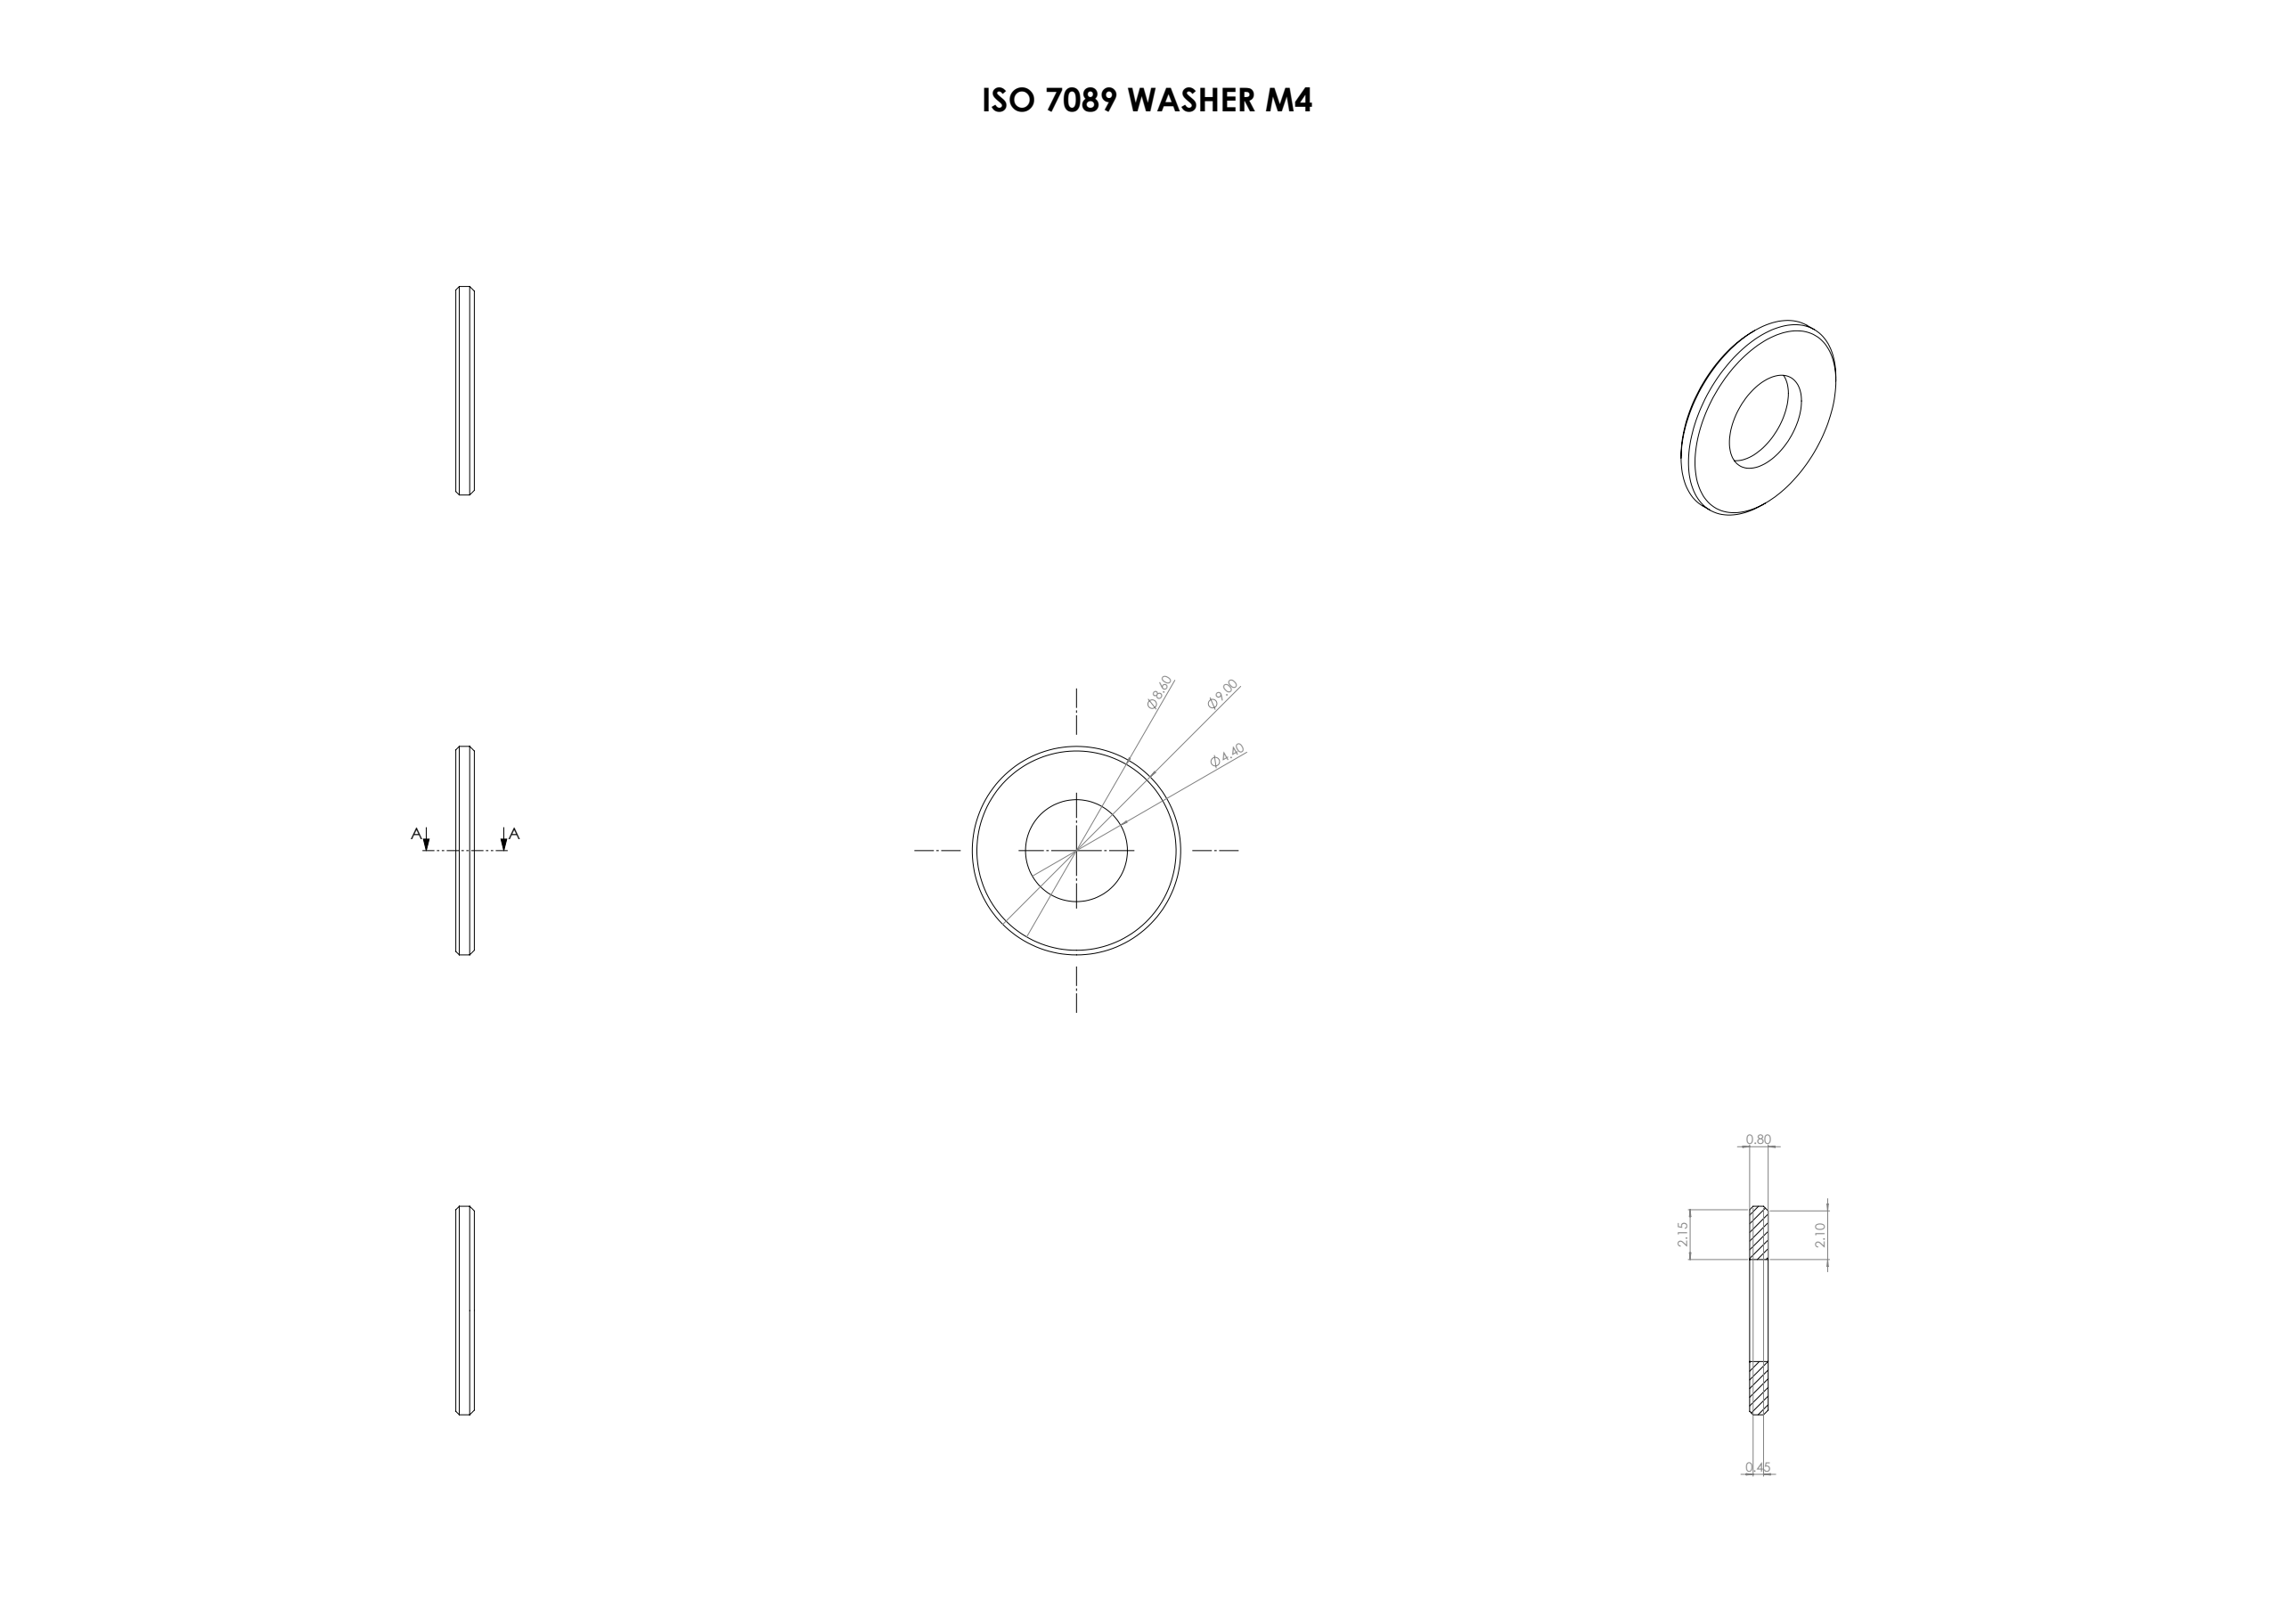
ISO-10303-21;
HEADER;
/* Generated by software containing ST-Developer
 * from STEP Tools, Inc. (www.steptools.com) 
 */

FILE_DESCRIPTION(
/* description */ (''),
/* implementation_level */ '2;1');

FILE_NAME(
/* name */ '12_ISO_7089_Washer_M4.step',
/* time_stamp */ '2026-10-21T02:01:14-07:00',
/* author */ (''),
/* organization */ (''),
/* preprocessor_version */ 'ST-DEVELOPER v20.2',
/* originating_system */ 'Autodesk Translation Framework v15.15.0.0',
/* authorisation */ '');

FILE_SCHEMA (('AUTOMOTIVE_DESIGN { 1 0 10303 214 3 1 1 }'));
ENDSEC;

DATA;
#10=MECHANICAL_DESIGN_GEOMETRIC_PRESENTATION_REPRESENTATION('',(#624),#37181);
#598=SHAPE_REPRESENTATION_RELATIONSHIP('SRR','None',#37248,#611);
#611=ADVANCED_BREP_SHAPE_REPRESENTATION('',(#637),#37178);
#624=STYLED_ITEM('',(#37380),#637);
#637=MANIFOLD_SOLID_BREP('Body1',#14786);
#684=FACE_BOUND('',#3017,.T.);
#685=FACE_BOUND('',#3020,.T.);
#910=CYLINDRICAL_SURFACE('',#16004,4.5);
#911=CYLINDRICAL_SURFACE('',#16008,2.2);
#1258=CIRCLE('',#16001,4.3);
#1259=CIRCLE('',#16002,4.5);
#1260=CIRCLE('',#16003,4.5);
#1261=CIRCLE('',#16005,4.5);
#1262=CIRCLE('',#16007,2.2);
#1263=CIRCLE('',#16009,2.2);
#1264=CIRCLE('',#16011,4.35);
#1360=CONICAL_SURFACE('',#16000,4.4,0.785398163397449);
#1361=CONICAL_SURFACE('',#16012,4.425,0.785398163397451);
#2130=FACE_OUTER_BOUND('',#3014,.T.);
#2131=FACE_OUTER_BOUND('',#3015,.T.);
#2132=FACE_OUTER_BOUND('',#3016,.T.);
#2133=FACE_OUTER_BOUND('',#3018,.T.);
#2134=FACE_OUTER_BOUND('',#3019,.T.);
#2135=FACE_OUTER_BOUND('',#3021,.T.);
#3014=EDGE_LOOP('',(#13047,#13048,#13049,#13050,#13051));
#3015=EDGE_LOOP('',(#13052,#13053,#13054,#13055,#13056));
#3016=EDGE_LOOP('',(#13057));
#3017=EDGE_LOOP('',(#13058));
#3018=EDGE_LOOP('',(#13059,#13060,#13061,#13062));
#3019=EDGE_LOOP('',(#13063));
#3020=EDGE_LOOP('',(#13064));
#3021=EDGE_LOOP('',(#13065,#13066,#13067,#13068));
#4371=LINE('',#34284,#5610);
#4372=LINE('',#34290,#5611);
#4373=LINE('',#34297,#5612);
#4374=LINE('',#34303,#5613);
#5610=VECTOR('',#19431,4.4);
#5611=VECTOR('',#19438,4.5);
#5612=VECTOR('',#19447,2.2);
#5613=VECTOR('',#19456,4.425);
#6891=VERTEX_POINT('',#34281);
#6892=VERTEX_POINT('',#34283);
#6893=VERTEX_POINT('',#34285);
#6894=VERTEX_POINT('',#34289);
#6895=VERTEX_POINT('',#34293);
#6896=VERTEX_POINT('',#34296);
#6897=VERTEX_POINT('',#34300);
#8965=EDGE_CURVE('',#6891,#6891,#1258,.T.);
#8966=EDGE_CURVE('',#6891,#6892,#4371,.T.);
#8967=EDGE_CURVE('',#6892,#6893,#1259,.T.);
#8968=EDGE_CURVE('',#6893,#6892,#1260,.T.);
#8969=EDGE_CURVE('',#6893,#6894,#4372,.T.);
#8970=EDGE_CURVE('',#6894,#6894,#1261,.T.);
#8971=EDGE_CURVE('',#6895,#6895,#1262,.T.);
#8972=EDGE_CURVE('',#6895,#6896,#4373,.T.);
#8973=EDGE_CURVE('',#6896,#6896,#1263,.T.);
#8974=EDGE_CURVE('',#6897,#6897,#1264,.T.);
#8975=EDGE_CURVE('',#6894,#6897,#4374,.T.);
#13047=ORIENTED_EDGE('',*,*,#8965,.T.);
#13048=ORIENTED_EDGE('',*,*,#8966,.T.);
#13049=ORIENTED_EDGE('',*,*,#8967,.T.);
#13050=ORIENTED_EDGE('',*,*,#8968,.T.);
#13051=ORIENTED_EDGE('',*,*,#8966,.F.);
#13052=ORIENTED_EDGE('',*,*,#8967,.F.);
#13053=ORIENTED_EDGE('',*,*,#8968,.F.);
#13054=ORIENTED_EDGE('',*,*,#8969,.T.);
#13055=ORIENTED_EDGE('',*,*,#8970,.T.);
#13056=ORIENTED_EDGE('',*,*,#8969,.F.);
#13057=ORIENTED_EDGE('',*,*,#8965,.F.);
#13058=ORIENTED_EDGE('',*,*,#8971,.F.);
#13059=ORIENTED_EDGE('',*,*,#8971,.T.);
#13060=ORIENTED_EDGE('',*,*,#8972,.T.);
#13061=ORIENTED_EDGE('',*,*,#8973,.F.);
#13062=ORIENTED_EDGE('',*,*,#8972,.F.);
#13063=ORIENTED_EDGE('',*,*,#8974,.F.);
#13064=ORIENTED_EDGE('',*,*,#8973,.T.);
#13065=ORIENTED_EDGE('',*,*,#8970,.F.);
#13066=ORIENTED_EDGE('',*,*,#8975,.T.);
#13067=ORIENTED_EDGE('',*,*,#8974,.T.);
#13068=ORIENTED_EDGE('',*,*,#8975,.F.);
#13910=PLANE('',#16006);
#13911=PLANE('',#16010);
#14698=ADVANCED_FACE('',(#2130),#1360,.T.);
#14699=ADVANCED_FACE('',(#2131),#910,.T.);
#14700=ADVANCED_FACE('',(#2132,#684),#13910,.T.);
#14701=ADVANCED_FACE('',(#2133),#911,.F.);
#14702=ADVANCED_FACE('',(#2134,#685),#13911,.T.);
#14703=ADVANCED_FACE('',(#2135),#1361,.T.);
#14786=CLOSED_SHELL('',(#14698,#14699,#14700,#14701,#14702,#14703));
#15999=AXIS2_PLACEMENT_3D('',#34279,#19425,#19426);
#16000=AXIS2_PLACEMENT_3D('',#34280,#19427,#19428);
#16001=AXIS2_PLACEMENT_3D('',#34282,#19429,#19430);
#16002=AXIS2_PLACEMENT_3D('',#34286,#19432,#19433);
#16003=AXIS2_PLACEMENT_3D('',#34287,#19434,#19435);
#16004=AXIS2_PLACEMENT_3D('',#34288,#19436,#19437);
#16005=AXIS2_PLACEMENT_3D('',#34291,#19439,#19440);
#16006=AXIS2_PLACEMENT_3D('',#34292,#19441,#19442);
#16007=AXIS2_PLACEMENT_3D('',#34294,#19443,#19444);
#16008=AXIS2_PLACEMENT_3D('',#34295,#19445,#19446);
#16009=AXIS2_PLACEMENT_3D('',#34298,#19448,#19449);
#16010=AXIS2_PLACEMENT_3D('',#34299,#19450,#19451);
#16011=AXIS2_PLACEMENT_3D('',#34301,#19452,#19453);
#16012=AXIS2_PLACEMENT_3D('',#34302,#19454,#19455);
#19425=DIRECTION('axis',(0.,0.,1.));
#19426=DIRECTION('refdir',(1.,0.,0.));
#19427=DIRECTION('center_axis',(-1.,0.,0.));
#19428=DIRECTION('ref_axis',(0.,-1.,0.));
#19429=DIRECTION('center_axis',(-1.,0.,0.));
#19430=DIRECTION('ref_axis',(0.,-1.,0.));
#19431=DIRECTION('',(-0.707106781186547,0.707106781186548,8.65956056235494E-17));
#19432=DIRECTION('center_axis',(1.,0.,0.));
#19433=DIRECTION('ref_axis',(0.,-1.,0.));
#19434=DIRECTION('center_axis',(1.,0.,0.));
#19435=DIRECTION('ref_axis',(0.,-1.,0.));
#19436=DIRECTION('center_axis',(1.,0.,0.));
#19437=DIRECTION('ref_axis',(0.,1.,0.));
#19438=DIRECTION('',(-1.,0.,0.));
#19439=DIRECTION('center_axis',(1.,0.,0.));
#19440=DIRECTION('ref_axis',(0.,0.,-1.));
#19441=DIRECTION('center_axis',(1.,0.,0.));
#19442=DIRECTION('ref_axis',(0.,0.,-1.));
#19443=DIRECTION('center_axis',(1.,0.,0.));
#19444=DIRECTION('ref_axis',(0.,0.,-1.));
#19445=DIRECTION('center_axis',(1.,0.,0.));
#19446=DIRECTION('ref_axis',(0.,1.,0.));
#19447=DIRECTION('',(-1.,0.,0.));
#19448=DIRECTION('center_axis',(1.,0.,0.));
#19449=DIRECTION('ref_axis',(0.,0.,-1.));
#19450=DIRECTION('center_axis',(-1.,0.,0.));
#19451=DIRECTION('ref_axis',(0.,0.,1.));
#19452=DIRECTION('center_axis',(1.,0.,0.));
#19453=DIRECTION('ref_axis',(0.,0.,-1.));
#19454=DIRECTION('center_axis',(1.,0.,0.));
#19455=DIRECTION('ref_axis',(0.,1.,0.));
#19456=DIRECTION('',(-0.707106781186546,0.707106781186549,8.65956056235496E-17));
#34279=CARTESIAN_POINT('',(0.,0.,0.));
#34280=CARTESIAN_POINT('Origin',(0.7,0.,0.));
#34281=CARTESIAN_POINT('',(0.8,4.3,-5.26598123633362E-16));
#34282=CARTESIAN_POINT('Origin',(0.8,0.,0.));
#34283=CARTESIAN_POINT('',(0.6,4.5,5.51091059616309E-16));
#34284=CARTESIAN_POINT('',(0.7,4.4,5.38844591624835E-16));
#34285=CARTESIAN_POINT('',(0.6,-4.5,-5.51091059616309E-16));
#34286=CARTESIAN_POINT('Origin',(0.6,0.,0.));
#34287=CARTESIAN_POINT('Origin',(0.6,0.,0.));
#34288=CARTESIAN_POINT('Origin',(0.475,0.,0.));
#34289=CARTESIAN_POINT('',(0.15,-4.5,-5.51091059616309E-16));
#34290=CARTESIAN_POINT('',(0.475,-4.5,-5.51091059616309E-16));
#34291=CARTESIAN_POINT('Origin',(0.15,0.,0.));
#34292=CARTESIAN_POINT('Origin',(0.8,2.2,0.));
#34293=CARTESIAN_POINT('',(0.8,-2.2,-2.69422295812418E-16));
#34294=CARTESIAN_POINT('Origin',(0.8,0.,0.));
#34295=CARTESIAN_POINT('Origin',(0.4,0.,0.));
#34296=CARTESIAN_POINT('',(0.,-2.2,-2.69422295812418E-16));
#34297=CARTESIAN_POINT('',(0.4,-2.2,-2.69422295812418E-16));
#34298=CARTESIAN_POINT('Origin',(0.,0.,0.));
#34299=CARTESIAN_POINT('Origin',(0.,4.35,0.));
#34300=CARTESIAN_POINT('',(-3.20923843055709E-16,-4.35,-5.32721357629099E-16));
#34301=CARTESIAN_POINT('Origin',(0.,0.,0.));
#34302=CARTESIAN_POINT('Origin',(0.0749999999999999,0.,0.));
#34303=CARTESIAN_POINT('',(0.0749999999999999,-4.425,-5.41906208622704E-16));
#37163=UNCERTAINTY_MEASURE_WITH_UNIT(LENGTH_MEASURE(0.01),#37182,
'DISTANCE_ACCURACY_VALUE',
'Maximum model space distance between geometric entities at asserted c
onnectivities');
#37166=UNCERTAINTY_MEASURE_WITH_UNIT(LENGTH_MEASURE(0.01),#37182,
'DISTANCE_ACCURACY_VALUE',
'Maximum model space distance between geometric entities at asserted c
onnectivities');
#37178=(
GEOMETRIC_REPRESENTATION_CONTEXT(3)
GLOBAL_UNCERTAINTY_ASSIGNED_CONTEXT((#37163))
GLOBAL_UNIT_ASSIGNED_CONTEXT((#37182,#37184,#37185))
REPRESENTATION_CONTEXT('','3D')
);
#37181=(
GEOMETRIC_REPRESENTATION_CONTEXT(3)
GLOBAL_UNCERTAINTY_ASSIGNED_CONTEXT((#37166))
GLOBAL_UNIT_ASSIGNED_CONTEXT((#37182,#37184,#37185))
REPRESENTATION_CONTEXT('','3D')
);
#37182=(
LENGTH_UNIT()
NAMED_UNIT(*)
SI_UNIT(.MILLI.,.METRE.)
);
#37184=(
NAMED_UNIT(*)
PLANE_ANGLE_UNIT()
SI_UNIT($,.RADIAN.)
);
#37185=(
NAMED_UNIT(*)
SI_UNIT($,.STERADIAN.)
SOLID_ANGLE_UNIT()
);
#37197=SHAPE_DEFINITION_REPRESENTATION(#37211,#37248);
#37211=PRODUCT_DEFINITION_SHAPE('',$,#37263);
#37248=SHAPE_REPRESENTATION('',(#15999),#37178);
#37251=PRODUCT_DEFINITION_CONTEXT('part definition',#37295,'design');
#37263=PRODUCT_DEFINITION('2026-10-20-13-24-04-900',
'12_ISO_7089_Washer_M4',#37277,#37251);
#37277=PRODUCT_DEFINITION_FORMATION('',$,#37308);
#37295=APPLICATION_CONTEXT(
'Core Data for Automotive Mechanical Design Process');
#37296=PRODUCT_CONTEXT('part definition',#37295,'mechanical');
#37308=PRODUCT('2026-10-20-13-24-04-900','12_ISO_7089_Washer_M4',$,(#37296));
#37374=COLOUR_RGB('Black',0.12,0.14,0.17);
#37375=FILL_AREA_STYLE_COLOUR('',#37374);
#37376=FILL_AREA_STYLE('',(#37375));
#37377=SURFACE_STYLE_FILL_AREA(#37376);
#37378=SURFACE_SIDE_STYLE('',(#37377));
#37379=SURFACE_STYLE_USAGE(.BOTH.,#37378);
#37380=PRESENTATION_STYLE_ASSIGNMENT((#37379));
ENDSEC;
END-ISO-10303-21;
